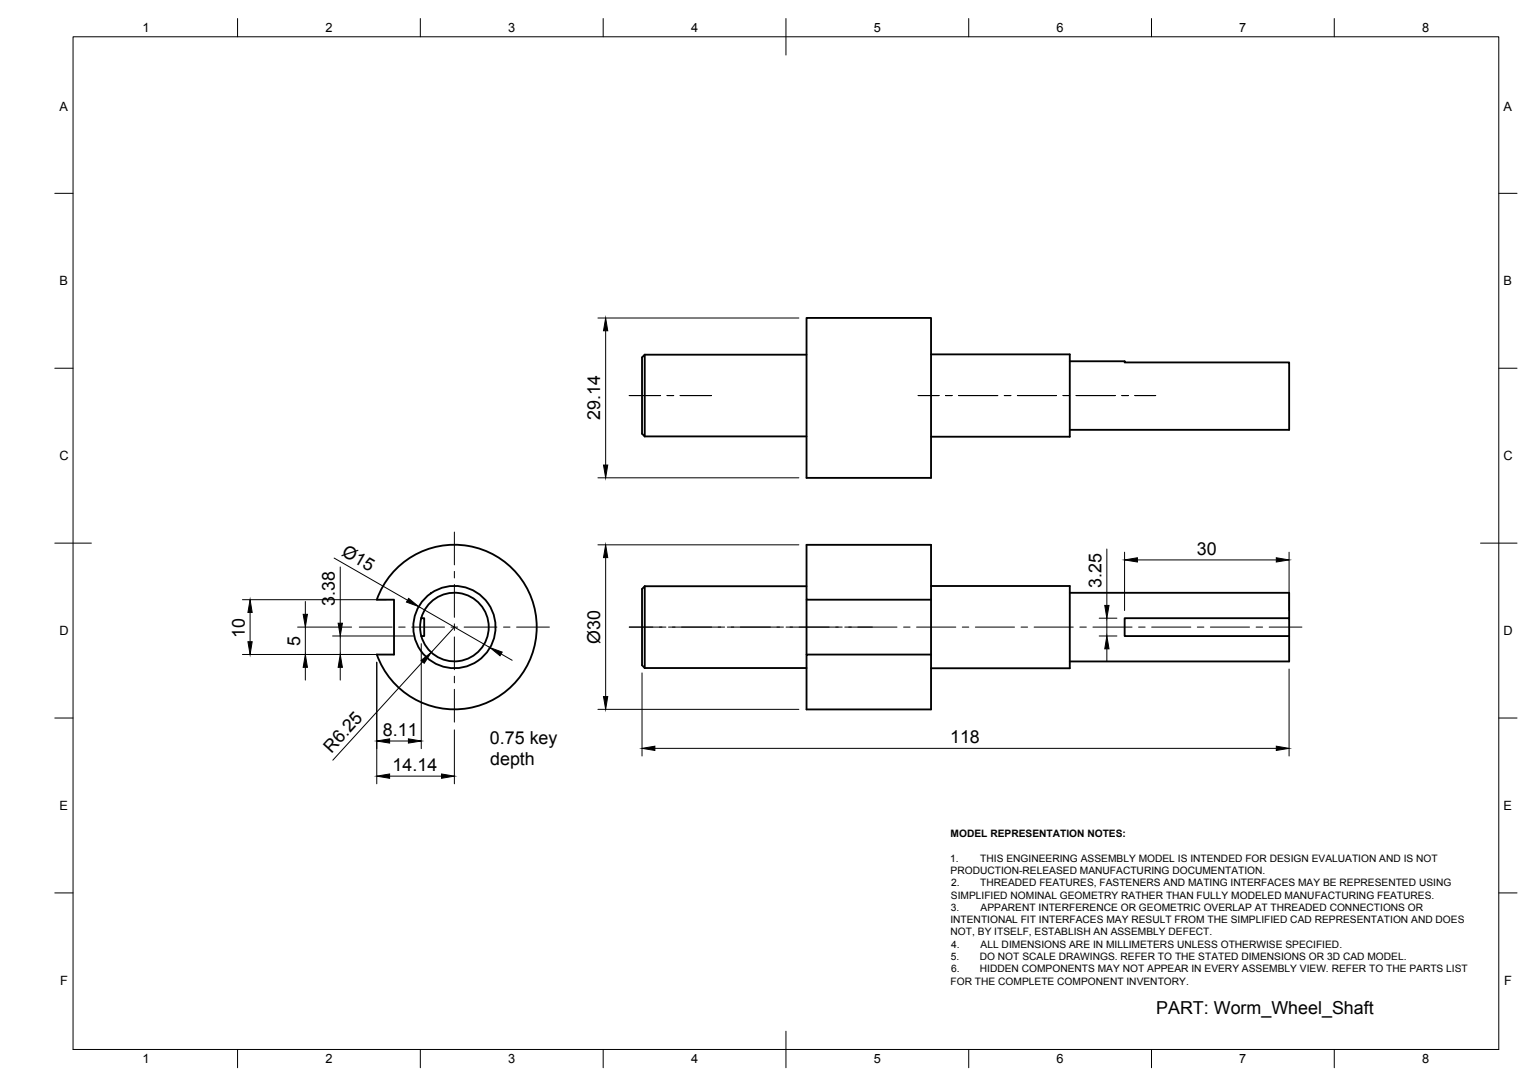
ISO-10303-21;
HEADER;
/* Generated by software containing ST-Developer
 * from STEP Tools, Inc. (www.steptools.com) 
 */

FILE_DESCRIPTION(
/* description */ ('STEP AP214'),
/* implementation_level */ '2;1');

FILE_NAME(
/* name */ 'Worm_Wheel_Shaft.step',
/* time_stamp */ '2026-10-05T13:15:56-07:00',
/* author */ (''),
/* organization */ (''),
/* preprocessor_version */ 'ST-DEVELOPER v20.2',
/* originating_system */ 'Autodesk Translation Framework v15.15.0.0',
/* authorisation */ '');

FILE_SCHEMA (('AUTOMOTIVE_DESIGN { 1 0 10303 214 3 1 1 }'));
ENDSEC;

DATA;
#10=MECHANICAL_DESIGN_GEOMETRIC_PRESENTATION_REPRESENTATION('',(#1347),#37881);
#593=CONICAL_SURFACE('',#11081,6.95000000000004,0.785398163397436);
#1323=SHAPE_REPRESENTATION_RELATIONSHIP('SRR','None',#37956,#1335);
#1335=ADVANCED_BREP_SHAPE_REPRESENTATION('',(#1359),#37871);
#1347=STYLED_ITEM('',(#38023),#1359);
#1359=MANIFOLD_SOLID_BREP('Body1',#10821);
#1402=FACE_BOUND('',#2276,.T.);
#1403=FACE_BOUND('',#2278,.T.);
#1404=FACE_BOUND('',#2280,.T.);
#1492=PLANE('',#11098);
#1493=PLANE('',#11099);
#1494=PLANE('',#11100);
#1495=PLANE('',#11101);
#1496=PLANE('',#11102);
#1497=PLANE('',#11103);
#1498=PLANE('',#11104);
#1499=PLANE('',#11105);
#1500=PLANE('',#11106);
#1501=PLANE('',#11107);
#1502=PLANE('',#11108);
#1503=PLANE('',#11109);
#1631=FACE_OUTER_BOUND('',#2265,.T.);
#1632=FACE_OUTER_BOUND('',#2266,.T.);
#1633=FACE_OUTER_BOUND('',#2267,.T.);
#1634=FACE_OUTER_BOUND('',#2268,.T.);
#1635=FACE_OUTER_BOUND('',#2269,.T.);
#1636=FACE_OUTER_BOUND('',#2270,.T.);
#1637=FACE_OUTER_BOUND('',#2271,.T.);
#1638=FACE_OUTER_BOUND('',#2272,.T.);
#1639=FACE_OUTER_BOUND('',#2273,.T.);
#1640=FACE_OUTER_BOUND('',#2274,.T.);
#1641=FACE_OUTER_BOUND('',#2275,.T.);
#1642=FACE_OUTER_BOUND('',#2277,.T.);
#1643=FACE_OUTER_BOUND('',#2279,.T.);
#1644=FACE_OUTER_BOUND('',#2281,.T.);
#1645=FACE_OUTER_BOUND('',#2282,.T.);
#1646=FACE_OUTER_BOUND('',#2283,.T.);
#1647=FACE_OUTER_BOUND('',#2284,.T.);
#2265=EDGE_LOOP('',(#7067,#7068,#7069,#7070,#7071));
#2266=EDGE_LOOP('',(#7072,#7073,#7074,#7075));
#2267=EDGE_LOOP('',(#7076,#7077,#7078,#7079));
#2268=EDGE_LOOP('',(#7080,#7081,#7082,#7083,#7084));
#2269=EDGE_LOOP('',(#7085,#7086,#7087,#7088,#7089,#7090,#7091,#7092));
#2270=EDGE_LOOP('',(#7093,#7094,#7095,#7096,#7097));
#2271=EDGE_LOOP('',(#7098));
#2272=EDGE_LOOP('',(#7099,#7100,#7101,#7102));
#2273=EDGE_LOOP('',(#7103,#7104,#7105,#7106));
#2274=EDGE_LOOP('',(#7107,#7108,#7109,#7110));
#2275=EDGE_LOOP('',(#7111,#7112,#7113,#7114));
#2276=EDGE_LOOP('',(#7115));
#2277=EDGE_LOOP('',(#7116,#7117,#7118,#7119));
#2278=EDGE_LOOP('',(#7120));
#2279=EDGE_LOOP('',(#7121));
#2280=EDGE_LOOP('',(#7122));
#2281=EDGE_LOOP('',(#7123,#7124,#7125,#7126));
#2282=EDGE_LOOP('',(#7127,#7128,#7129,#7130));
#2283=EDGE_LOOP('',(#7131,#7132,#7133,#7134));
#2284=EDGE_LOOP('',(#7135,#7136,#7137,#7138));
#2965=LINE('',#17230,#3266);
#2966=LINE('',#17236,#3267);
#2967=LINE('',#17243,#3268);
#2968=LINE('',#17246,#3269);
#2969=LINE('',#17249,#3270);
#2970=LINE('',#17255,#3271);
#2971=LINE('',#17259,#3272);
#2972=LINE('',#17263,#3273);
#2973=LINE('',#17268,#3274);
#2974=LINE('',#17269,#3275);
#2975=LINE('',#17270,#3276);
#2976=LINE('',#17274,#3277);
#2977=LINE('',#17276,#3278);
#2978=LINE('',#17277,#3279);
#2979=LINE('',#17280,#3280);
#2980=LINE('',#17282,#3281);
#2981=LINE('',#17283,#3282);
#2982=LINE('',#17285,#3283);
#2983=LINE('',#17286,#3284);
#2984=LINE('',#17292,#3285);
#2985=LINE('',#17294,#3286);
#2986=LINE('',#17295,#3287);
#2987=LINE('',#17297,#3288);
#2988=LINE('',#17299,#3289);
#3266=VECTOR('',#12224,6.95000000000004);
#3267=VECTOR('',#12231,7.5);
#3268=VECTOR('',#12238,1000.);
#3269=VECTOR('',#12241,1000.);
#3270=VECTOR('',#12244,7.45);
#3271=VECTOR('',#12251,6.25);
#3272=VECTOR('',#12254,1000.);
#3273=VECTOR('',#12257,1000.);
#3274=VECTOR('',#12262,1000.);
#3275=VECTOR('',#12263,1000.);
#3276=VECTOR('',#12264,1000.);
#3277=VECTOR('',#12269,1000.);
#3278=VECTOR('',#12270,1000.);
#3279=VECTOR('',#12271,1000.);
#3280=VECTOR('',#12274,1000.);
#3281=VECTOR('',#12275,1000.);
#3282=VECTOR('',#12276,1000.);
#3283=VECTOR('',#12279,1000.);
#3284=VECTOR('',#12280,1000.);
#3285=VECTOR('',#12289,1000.);
#3286=VECTOR('',#12290,1000.);
#3287=VECTOR('',#12291,1000.);
#3288=VECTOR('',#12294,1000.);
#3289=VECTOR('',#12297,1000.);
#3522=CIRCLE('',#11082,7.45);
#3523=CIRCLE('',#11083,7.45);
#3524=CIRCLE('',#11084,6.95000000000004);
#3525=CIRCLE('',#11086,7.5);
#3526=CIRCLE('',#11087,7.5);
#3527=CIRCLE('',#11089,15.);
#3528=CIRCLE('',#11090,15.);
#3529=CIRCLE('',#11092,7.45);
#3530=CIRCLE('',#11094,6.25);
#3531=CIRCLE('',#11095,6.25);
#3532=CIRCLE('',#11096,6.25);
#3533=CIRCLE('',#11097,6.25);
#4110=VERTEX_POINT('',#17225);
#4111=VERTEX_POINT('',#17226);
#4112=VERTEX_POINT('',#17229);
#4113=VERTEX_POINT('',#17233);
#4114=VERTEX_POINT('',#17235);
#4115=VERTEX_POINT('',#17239);
#4116=VERTEX_POINT('',#17240);
#4117=VERTEX_POINT('',#17242);
#4118=VERTEX_POINT('',#17244);
#4119=VERTEX_POINT('',#17248);
#4120=VERTEX_POINT('',#17252);
#4121=VERTEX_POINT('',#17254);
#4122=VERTEX_POINT('',#17256);
#4123=VERTEX_POINT('',#17258);
#4124=VERTEX_POINT('',#17260);
#4125=VERTEX_POINT('',#17262);
#4126=VERTEX_POINT('',#17266);
#4127=VERTEX_POINT('',#17267);
#4128=VERTEX_POINT('',#17273);
#4129=VERTEX_POINT('',#17275);
#4130=VERTEX_POINT('',#17279);
#4131=VERTEX_POINT('',#17281);
#4132=VERTEX_POINT('',#17291);
#4133=VERTEX_POINT('',#17293);
#5244=EDGE_CURVE('',#4110,#4111,#3522,.T.);
#5245=EDGE_CURVE('',#4111,#4110,#3523,.T.);
#5246=EDGE_CURVE('',#4111,#4112,#2965,.T.);
#5247=EDGE_CURVE('',#4112,#4112,#3524,.T.);
#5248=EDGE_CURVE('',#4113,#4113,#3525,.T.);
#5249=EDGE_CURVE('',#4113,#4114,#2966,.T.);
#5250=EDGE_CURVE('',#4114,#4114,#3526,.T.);
#5251=EDGE_CURVE('',#4115,#4116,#3527,.T.);
#5252=EDGE_CURVE('',#4115,#4117,#2967,.T.);
#5253=EDGE_CURVE('',#4117,#4118,#3528,.T.);
#5254=EDGE_CURVE('',#4116,#4118,#2968,.T.);
#5255=EDGE_CURVE('',#4110,#4119,#2969,.T.);
#5256=EDGE_CURVE('',#4119,#4119,#3529,.T.);
#5257=EDGE_CURVE('',#4120,#4120,#3530,.T.);
#5258=EDGE_CURVE('',#4120,#4121,#2970,.T.);
#5259=EDGE_CURVE('',#4122,#4121,#3531,.T.);
#5260=EDGE_CURVE('',#4123,#4122,#2971,.T.);
#5261=EDGE_CURVE('',#4124,#4123,#3532,.T.);
#5262=EDGE_CURVE('',#4124,#4125,#2972,.T.);
#5263=EDGE_CURVE('',#4121,#4125,#3533,.T.);
#5264=EDGE_CURVE('',#4126,#4127,#2973,.T.);
#5265=EDGE_CURVE('',#4126,#4122,#2974,.T.);
#5266=EDGE_CURVE('',#4127,#4125,#2975,.T.);
#5267=EDGE_CURVE('',#4128,#4117,#2976,.T.);
#5268=EDGE_CURVE('',#4129,#4115,#2977,.T.);
#5269=EDGE_CURVE('',#4129,#4128,#2978,.T.);
#5270=EDGE_CURVE('',#4130,#4118,#2979,.T.);
#5271=EDGE_CURVE('',#4131,#4130,#2980,.T.);
#5272=EDGE_CURVE('',#4131,#4116,#2981,.T.);
#5273=EDGE_CURVE('',#4128,#4130,#2982,.T.);
#5274=EDGE_CURVE('',#4129,#4131,#2983,.T.);
#5275=EDGE_CURVE('',#4132,#4123,#2984,.T.);
#5276=EDGE_CURVE('',#4132,#4133,#2985,.T.);
#5277=EDGE_CURVE('',#4133,#4124,#2986,.T.);
#5278=EDGE_CURVE('',#4132,#4126,#2987,.T.);
#5279=EDGE_CURVE('',#4133,#4127,#2988,.T.);
#7067=ORIENTED_EDGE('',*,*,#5244,.F.);
#7068=ORIENTED_EDGE('',*,*,#5245,.F.);
#7069=ORIENTED_EDGE('',*,*,#5246,.T.);
#7070=ORIENTED_EDGE('',*,*,#5247,.F.);
#7071=ORIENTED_EDGE('',*,*,#5246,.F.);
#7072=ORIENTED_EDGE('',*,*,#5248,.T.);
#7073=ORIENTED_EDGE('',*,*,#5249,.T.);
#7074=ORIENTED_EDGE('',*,*,#5250,.F.);
#7075=ORIENTED_EDGE('',*,*,#5249,.F.);
#7076=ORIENTED_EDGE('',*,*,#5251,.F.);
#7077=ORIENTED_EDGE('',*,*,#5252,.T.);
#7078=ORIENTED_EDGE('',*,*,#5253,.T.);
#7079=ORIENTED_EDGE('',*,*,#5254,.F.);
#7080=ORIENTED_EDGE('',*,*,#5244,.T.);
#7081=ORIENTED_EDGE('',*,*,#5245,.T.);
#7082=ORIENTED_EDGE('',*,*,#5255,.T.);
#7083=ORIENTED_EDGE('',*,*,#5256,.T.);
#7084=ORIENTED_EDGE('',*,*,#5255,.F.);
#7085=ORIENTED_EDGE('',*,*,#5257,.T.);
#7086=ORIENTED_EDGE('',*,*,#5258,.T.);
#7087=ORIENTED_EDGE('',*,*,#5259,.F.);
#7088=ORIENTED_EDGE('',*,*,#5260,.F.);
#7089=ORIENTED_EDGE('',*,*,#5261,.F.);
#7090=ORIENTED_EDGE('',*,*,#5262,.T.);
#7091=ORIENTED_EDGE('',*,*,#5263,.F.);
#7092=ORIENTED_EDGE('',*,*,#5258,.F.);
#7093=ORIENTED_EDGE('',*,*,#5264,.F.);
#7094=ORIENTED_EDGE('',*,*,#5265,.T.);
#7095=ORIENTED_EDGE('',*,*,#5259,.T.);
#7096=ORIENTED_EDGE('',*,*,#5263,.T.);
#7097=ORIENTED_EDGE('',*,*,#5266,.F.);
#7098=ORIENTED_EDGE('',*,*,#5247,.T.);
#7099=ORIENTED_EDGE('',*,*,#5267,.T.);
#7100=ORIENTED_EDGE('',*,*,#5252,.F.);
#7101=ORIENTED_EDGE('',*,*,#5268,.F.);
#7102=ORIENTED_EDGE('',*,*,#5269,.T.);
#7103=ORIENTED_EDGE('',*,*,#5270,.F.);
#7104=ORIENTED_EDGE('',*,*,#5271,.F.);
#7105=ORIENTED_EDGE('',*,*,#5272,.T.);
#7106=ORIENTED_EDGE('',*,*,#5254,.T.);
#7107=ORIENTED_EDGE('',*,*,#5273,.F.);
#7108=ORIENTED_EDGE('',*,*,#5269,.F.);
#7109=ORIENTED_EDGE('',*,*,#5274,.T.);
#7110=ORIENTED_EDGE('',*,*,#5271,.T.);
#7111=ORIENTED_EDGE('',*,*,#5268,.T.);
#7112=ORIENTED_EDGE('',*,*,#5251,.T.);
#7113=ORIENTED_EDGE('',*,*,#5272,.F.);
#7114=ORIENTED_EDGE('',*,*,#5274,.F.);
#7115=ORIENTED_EDGE('',*,*,#5248,.F.);
#7116=ORIENTED_EDGE('',*,*,#5267,.F.);
#7117=ORIENTED_EDGE('',*,*,#5273,.T.);
#7118=ORIENTED_EDGE('',*,*,#5270,.T.);
#7119=ORIENTED_EDGE('',*,*,#5253,.F.);
#7120=ORIENTED_EDGE('',*,*,#5256,.F.);
#7121=ORIENTED_EDGE('',*,*,#5250,.T.);
#7122=ORIENTED_EDGE('',*,*,#5257,.F.);
#7123=ORIENTED_EDGE('',*,*,#5261,.T.);
#7124=ORIENTED_EDGE('',*,*,#5275,.F.);
#7125=ORIENTED_EDGE('',*,*,#5276,.T.);
#7126=ORIENTED_EDGE('',*,*,#5277,.T.);
#7127=ORIENTED_EDGE('',*,*,#5260,.T.);
#7128=ORIENTED_EDGE('',*,*,#5265,.F.);
#7129=ORIENTED_EDGE('',*,*,#5278,.F.);
#7130=ORIENTED_EDGE('',*,*,#5275,.T.);
#7131=ORIENTED_EDGE('',*,*,#5277,.F.);
#7132=ORIENTED_EDGE('',*,*,#5279,.T.);
#7133=ORIENTED_EDGE('',*,*,#5266,.T.);
#7134=ORIENTED_EDGE('',*,*,#5262,.F.);
#7135=ORIENTED_EDGE('',*,*,#5264,.T.);
#7136=ORIENTED_EDGE('',*,*,#5279,.F.);
#7137=ORIENTED_EDGE('',*,*,#5276,.F.);
#7138=ORIENTED_EDGE('',*,*,#5278,.T.);
#10061=CYLINDRICAL_SURFACE('',#11085,7.5);
#10062=CYLINDRICAL_SURFACE('',#11088,15.);
#10063=CYLINDRICAL_SURFACE('',#11091,7.45);
#10064=CYLINDRICAL_SURFACE('',#11093,6.25);
#10276=ADVANCED_FACE('',(#1631),#593,.T.);
#10277=ADVANCED_FACE('',(#1632),#10061,.T.);
#10278=ADVANCED_FACE('',(#1633),#10062,.T.);
#10279=ADVANCED_FACE('',(#1634),#10063,.T.);
#10280=ADVANCED_FACE('',(#1635),#10064,.T.);
#10281=ADVANCED_FACE('',(#1636),#1492,.T.);
#10282=ADVANCED_FACE('',(#1637),#1493,.T.);
#10283=ADVANCED_FACE('',(#1638),#1494,.F.);
#10284=ADVANCED_FACE('',(#1639),#1495,.T.);
#10285=ADVANCED_FACE('',(#1640),#1496,.T.);
#10286=ADVANCED_FACE('',(#1641,#1402),#1497,.T.);
#10287=ADVANCED_FACE('',(#1642,#1403),#1498,.F.);
#10288=ADVANCED_FACE('',(#1643,#1404),#1499,.T.);
#10289=ADVANCED_FACE('',(#1644),#1500,.T.);
#10290=ADVANCED_FACE('',(#1645),#1501,.T.);
#10291=ADVANCED_FACE('',(#1646),#1502,.F.);
#10292=ADVANCED_FACE('',(#1647),#1503,.F.);
#10821=CLOSED_SHELL('',(#10276,#10277,#10278,#10279,#10280,#10281,#10282,
#10283,#10284,#10285,#10286,#10287,#10288,#10289,#10290,#10291,#10292));
#11080=AXIS2_PLACEMENT_3D('',#17223,#12216,#12217);
#11081=AXIS2_PLACEMENT_3D('',#17224,#12218,#12219);
#11082=AXIS2_PLACEMENT_3D('',#17227,#12220,#12221);
#11083=AXIS2_PLACEMENT_3D('',#17228,#12222,#12223);
#11084=AXIS2_PLACEMENT_3D('',#17231,#12225,#12226);
#11085=AXIS2_PLACEMENT_3D('',#17232,#12227,#12228);
#11086=AXIS2_PLACEMENT_3D('',#17234,#12229,#12230);
#11087=AXIS2_PLACEMENT_3D('',#17237,#12232,#12233);
#11088=AXIS2_PLACEMENT_3D('',#17238,#12234,#12235);
#11089=AXIS2_PLACEMENT_3D('',#17241,#12236,#12237);
#11090=AXIS2_PLACEMENT_3D('',#17245,#12239,#12240);
#11091=AXIS2_PLACEMENT_3D('',#17247,#12242,#12243);
#11092=AXIS2_PLACEMENT_3D('',#17250,#12245,#12246);
#11093=AXIS2_PLACEMENT_3D('',#17251,#12247,#12248);
#11094=AXIS2_PLACEMENT_3D('',#17253,#12249,#12250);
#11095=AXIS2_PLACEMENT_3D('',#17257,#12252,#12253);
#11096=AXIS2_PLACEMENT_3D('',#17261,#12255,#12256);
#11097=AXIS2_PLACEMENT_3D('',#17264,#12258,#12259);
#11098=AXIS2_PLACEMENT_3D('',#17265,#12260,#12261);
#11099=AXIS2_PLACEMENT_3D('',#17271,#12265,#12266);
#11100=AXIS2_PLACEMENT_3D('',#17272,#12267,#12268);
#11101=AXIS2_PLACEMENT_3D('',#17278,#12272,#12273);
#11102=AXIS2_PLACEMENT_3D('',#17284,#12277,#12278);
#11103=AXIS2_PLACEMENT_3D('',#17287,#12281,#12282);
#11104=AXIS2_PLACEMENT_3D('',#17288,#12283,#12284);
#11105=AXIS2_PLACEMENT_3D('',#17289,#12285,#12286);
#11106=AXIS2_PLACEMENT_3D('',#17290,#12287,#12288);
#11107=AXIS2_PLACEMENT_3D('',#17296,#12292,#12293);
#11108=AXIS2_PLACEMENT_3D('',#17298,#12295,#12296);
#11109=AXIS2_PLACEMENT_3D('',#17300,#12298,#12299);
#12216=DIRECTION('axis',(0.,0.,1.));
#12217=DIRECTION('refdir',(1.,0.,0.));
#12218=DIRECTION('center_axis',(1.,0.,5.91645678915759E-31));
#12219=DIRECTION('ref_axis',(5.91645678915759E-31,-1.28868988380477E-29,
-1.));
#12220=DIRECTION('center_axis',(1.,0.,5.91645678915759E-31));
#12221=DIRECTION('ref_axis',(-5.91645678915759E-31,1.29257043247465E-29,
1.));
#12222=DIRECTION('center_axis',(1.,0.,5.91645678915759E-31));
#12223=DIRECTION('ref_axis',(-5.91645678915759E-31,1.29257043247465E-29,
1.));
#12224=DIRECTION('',(-0.707106781186556,8.65956056235392E-17,-0.707106781186539));
#12225=DIRECTION('center_axis',(-1.,0.,-5.91645678915759E-31));
#12226=DIRECTION('ref_axis',(-5.91645678915759E-31,1.28868988380477E-29,
1.));
#12227=DIRECTION('center_axis',(-1.,0.,-5.91645678915759E-31));
#12228=DIRECTION('ref_axis',(-5.91645678915759E-31,1.29422492262822E-29,
1.));
#12229=DIRECTION('center_axis',(1.,0.,5.91645678915759E-31));
#12230=DIRECTION('ref_axis',(5.91645678915759E-31,-1.29422492262822E-29,
-1.));
#12231=DIRECTION('',(1.,0.,5.91645678915759E-31));
#12232=DIRECTION('center_axis',(1.,0.,5.91645678915759E-31));
#12233=DIRECTION('ref_axis',(5.91645678915759E-31,-1.29422492262822E-29,
-1.));
#12234=DIRECTION('center_axis',(-1.,0.,-5.91645678915759E-31));
#12235=DIRECTION('ref_axis',(7.00649232162409E-46,-1.,-1.07187543957222E-15));
#12236=DIRECTION('center_axis',(1.,0.,5.91645678915759E-31));
#12237=DIRECTION('ref_axis',(5.91645678915759E-31,-1.28395329625816E-29,
-1.));
#12238=DIRECTION('',(-1.,0.,-5.91645678915759E-31));
#12239=DIRECTION('center_axis',(1.,0.,5.91645678915759E-31));
#12240=DIRECTION('ref_axis',(5.91645678915759E-31,-1.28395329625816E-29,
-1.));
#12241=DIRECTION('',(-1.,0.,-5.91645678915759E-31));
#12242=DIRECTION('center_axis',(-1.,0.,-5.91645678915759E-31));
#12243=DIRECTION('ref_axis',(-5.91645678915759E-31,1.28868988380477E-29,
1.));
#12244=DIRECTION('',(1.,0.,5.91645678915759E-31));
#12245=DIRECTION('center_axis',(-1.,0.,-5.91645678915759E-31));
#12246=DIRECTION('ref_axis',(-5.91645678915759E-31,1.29257043247465E-29,
1.));
#12247=DIRECTION('center_axis',(-1.,0.,-5.91645678915759E-31));
#12248=DIRECTION('ref_axis',(-5.91645678915759E-31,1.28868988380477E-29,
1.));
#12249=DIRECTION('center_axis',(1.,0.,5.91645678915759E-31));
#12250=DIRECTION('ref_axis',(5.91645678915759E-31,-1.28189897098414E-29,
-1.));
#12251=DIRECTION('',(1.,0.,5.91645678915759E-31));
#12252=DIRECTION('center_axis',(1.,0.,5.91645678915759E-31));
#12253=DIRECTION('ref_axis',(5.91645678915759E-31,-1.28868988380477E-29,
-1.));
#12254=DIRECTION('',(1.,0.,5.91645678915759E-31));
#12255=DIRECTION('center_axis',(1.,0.,5.91645678915759E-31));
#12256=DIRECTION('ref_axis',(5.91645678915759E-31,-1.28189897098414E-29,
-1.));
#12257=DIRECTION('',(1.,0.,5.91645678915759E-31));
#12258=DIRECTION('center_axis',(1.,0.,5.91645678915759E-31));
#12259=DIRECTION('ref_axis',(5.91645678915759E-31,-1.28868988380477E-29,
-1.));
#12260=DIRECTION('center_axis',(1.,-1.52489560243109E-59,-5.91645678915759E-31));
#12261=DIRECTION('ref_axis',(-5.91645678915759E-31,-1.28868988380477E-29,
-1.));
#12262=DIRECTION('',(-3.94430452610506E-31,2.22044604925018E-16,-1.));
#12263=DIRECTION('',(0.,1.,1.28868988380477E-29));
#12264=DIRECTION('',(0.,1.,1.28868988380477E-29));
#12265=DIRECTION('center_axis',(-1.,1.52489560243109E-59,5.91645678915759E-31));
#12266=DIRECTION('ref_axis',(5.91645678915759E-31,1.28868988380477E-29,
1.));
#12267=DIRECTION('center_axis',(-5.91645678915759E-31,1.28868988380477E-29,
1.));
#12268=DIRECTION('ref_axis',(1.,5.52714787526044E-76,5.91645678915759E-31));
#12269=DIRECTION('',(0.,1.,1.28868988380477E-29));
#12270=DIRECTION('',(0.,1.,1.28868988380477E-29));
#12271=DIRECTION('',(-1.,0.,-5.91645678915759E-31));
#12272=DIRECTION('center_axis',(-5.91645678915759E-31,1.28868988380477E-29,
1.));
#12273=DIRECTION('ref_axis',(1.,5.52714787526044E-76,5.91645678915759E-31));
#12274=DIRECTION('',(0.,1.,1.28868988380477E-29));
#12275=DIRECTION('',(-1.,0.,-5.91645678915759E-31));
#12276=DIRECTION('',(0.,1.,1.28868988380477E-29));
#12277=DIRECTION('center_axis',(-1.52489560243109E-59,1.,-1.28868988380477E-29));
#12278=DIRECTION('ref_axis',(5.91645678915759E-31,1.28868988380477E-29,
1.));
#12279=DIRECTION('',(-5.91645678915759E-31,-1.28868988380477E-29,-1.));
#12280=DIRECTION('',(-5.91645678915759E-31,-1.28868988380477E-29,-1.));
#12281=DIRECTION('center_axis',(1.,-1.52489560243109E-59,-5.91645678915759E-31));
#12282=DIRECTION('ref_axis',(-5.91645678915759E-31,-1.28868988380477E-29,
-1.));
#12283=DIRECTION('center_axis',(1.,-1.52489560243109E-59,-5.91645678915759E-31));
#12284=DIRECTION('ref_axis',(-5.91645678915759E-31,-1.28868988380477E-29,
-1.));
#12285=DIRECTION('center_axis',(1.,-1.52489560243109E-59,-5.91645678915759E-31));
#12286=DIRECTION('ref_axis',(-5.91645678915759E-31,-1.28868988380477E-29,
-1.));
#12287=DIRECTION('center_axis',(1.,-1.52489560243109E-59,-5.91645678915759E-31));
#12288=DIRECTION('ref_axis',(-5.91645678915759E-31,-1.28868988380477E-29,
-1.));
#12289=DIRECTION('',(0.,1.,1.28868988380477E-29));
#12290=DIRECTION('',(-3.94430452610506E-31,2.22044604925018E-16,-1.));
#12291=DIRECTION('',(0.,1.,1.28868988380477E-29));
#12292=DIRECTION('center_axis',(5.91645678915759E-31,-1.28868988380477E-29,
-1.));
#12293=DIRECTION('ref_axis',(-1.,-5.52714787526044E-76,-5.91645678915759E-31));
#12294=DIRECTION('',(1.,0.,5.91645678915759E-31));
#12295=DIRECTION('center_axis',(5.91645678915759E-31,-1.28868988380477E-29,
-1.));
#12296=DIRECTION('ref_axis',(-1.,-5.52714787526044E-76,-5.91645678915759E-31));
#12297=DIRECTION('',(1.,0.,5.91645678915759E-31));
#12298=DIRECTION('center_axis',(1.01610171333826E-59,-1.,-2.22044604925018E-16));
#12299=DIRECTION('ref_axis',(-3.94430452610506E-31,2.22044604925018E-16,
-1.));
#17223=CARTESIAN_POINT('',(0.,0.,0.));
#17224=CARTESIAN_POINT('Origin',(0.,0.,0.));
#17225=CARTESIAN_POINT('',(0.499999999999973,9.12361865364679E-16,-7.45));
#17226=CARTESIAN_POINT('',(0.499999999999979,-9.12361865364683E-16,7.45000000000001));
#17227=CARTESIAN_POINT('Origin',(0.499999999999973,-6.93889390390723E-15,
5.20417042793042E-15));
#17228=CARTESIAN_POINT('Origin',(0.499999999999973,-6.93889390390723E-15,
5.20417042793042E-15));
#17229=CARTESIAN_POINT('',(-2.67390226427335E-16,-8.51129525407326E-16,
6.95000000000004));
#17230=CARTESIAN_POINT('',(-4.11193746846455E-30,-8.51129525407326E-16,
6.95000000000004));
#17231=CARTESIAN_POINT('Origin',(0.,0.,0.));
#17232=CARTESIAN_POINT('Origin',(78.,-8.67361737988404E-15,6.93889390390723E-15));
#17233=CARTESIAN_POINT('',(52.7,-9.59210247924465E-15,-7.49999999999999));
#17234=CARTESIAN_POINT('Origin',(52.7,-8.67361737988404E-15,6.93889390390723E-15));
#17235=CARTESIAN_POINT('',(78.,-9.59210247924465E-15,-7.49999999999999));
#17236=CARTESIAN_POINT('',(78.,-9.59210247924465E-15,-7.49999999999999));
#17237=CARTESIAN_POINT('Origin',(78.,-8.67361737988404E-15,6.93889390390723E-15));
#17238=CARTESIAN_POINT('Origin',(52.7,-8.67361737988404E-15,6.93889390390723E-15));
#17239=CARTESIAN_POINT('',(52.7,14.1421356237309,5.00000000000001));
#17240=CARTESIAN_POINT('',(52.7,14.1421356237309,-4.99999999999999));
#17241=CARTESIAN_POINT('Origin',(52.7,-8.67361737988404E-15,6.93889390390723E-15));
#17242=CARTESIAN_POINT('',(30.,14.1421356237309,5.00000000000001));
#17243=CARTESIAN_POINT('',(52.7,14.1421356237309,5.00000000000001));
#17244=CARTESIAN_POINT('',(30.,14.142135623731,-4.99999999999999));
#17245=CARTESIAN_POINT('Origin',(30.,-6.93889390390723E-15,6.93889390390723E-15));
#17246=CARTESIAN_POINT('',(52.7,14.1421356237309,-4.99999999999999));
#17247=CARTESIAN_POINT('Origin',(0.,0.,0.));
#17248=CARTESIAN_POINT('',(30.,-9.12361865364874E-16,-7.45));
#17249=CARTESIAN_POINT('',(4.4077603079224E-30,-9.12361865364874E-16,-7.45));
#17250=CARTESIAN_POINT('Origin',(30.,-6.93889390390723E-15,6.93889390390723E-15));
#17251=CARTESIAN_POINT('Origin',(118.,0.,0.));
#17252=CARTESIAN_POINT('',(78.,-7.65404249467176E-16,-6.25));
#17253=CARTESIAN_POINT('Origin',(78.,-8.67361737988404E-15,6.93889390390723E-15));
#17254=CARTESIAN_POINT('',(118.,-7.65404249467176E-16,-6.25));
#17255=CARTESIAN_POINT('',(118.,-7.65404249467176E-16,-6.25));
#17256=CARTESIAN_POINT('',(118.,6.03505385228666,1.625));
#17257=CARTESIAN_POINT('Origin',(118.,0.,0.));
#17258=CARTESIAN_POINT('',(88.,6.03505385228665,1.625));
#17259=CARTESIAN_POINT('',(118.,6.03505385228666,1.625));
#17260=CARTESIAN_POINT('',(88.,6.03505385228665,-1.625));
#17261=CARTESIAN_POINT('Origin',(88.,-6.93889390390723E-15,3.46944695195361E-15));
#17262=CARTESIAN_POINT('',(118.,6.03505385228666,-1.625));
#17263=CARTESIAN_POINT('',(118.,6.03505385228666,-1.625));
#17264=CARTESIAN_POINT('Origin',(118.,0.,0.));
#17265=CARTESIAN_POINT('Origin',(118.,0.,0.));
#17266=CARTESIAN_POINT('',(118.,5.5,1.625));
#17267=CARTESIAN_POINT('',(118.,5.5,-1.62499999999999));
#17268=CARTESIAN_POINT('',(118.,5.5,0.));
#17269=CARTESIAN_POINT('',(118.,-3.46944695195361E-15,1.625));
#17270=CARTESIAN_POINT('',(118.,-1.73472347597681E-15,-1.625));
#17271=CARTESIAN_POINT('Origin',(0.,0.,0.));
#17272=CARTESIAN_POINT('Origin',(52.7,-5.20417042793042E-15,5.00000000000001));
#17273=CARTESIAN_POINT('',(30.,11.,5.00000000000001));
#17274=CARTESIAN_POINT('',(30.,-6.93889390390723E-15,5.00000000000001));
#17275=CARTESIAN_POINT('',(52.7,11.,5.00000000000001));
#17276=CARTESIAN_POINT('',(52.7,-5.20417042793042E-15,5.00000000000001));
#17277=CARTESIAN_POINT('',(52.7,11.,5.00000000000001));
#17278=CARTESIAN_POINT('Origin',(52.7,-5.20417042793042E-15,-4.99999999999999));
#17279=CARTESIAN_POINT('',(30.,11.,-4.99999999999999));
#17280=CARTESIAN_POINT('',(30.,-5.20417042793042E-15,-4.99999999999999));
#17281=CARTESIAN_POINT('',(52.7,11.,-4.99999999999999));
#17282=CARTESIAN_POINT('',(52.7,11.,-4.99999999999999));
#17283=CARTESIAN_POINT('',(52.7,-5.20417042793042E-15,-4.99999999999999));
#17284=CARTESIAN_POINT('Origin',(52.7,11.,5.20417042793042E-15));
#17285=CARTESIAN_POINT('',(30.,11.,6.93889390390723E-15));
#17286=CARTESIAN_POINT('',(52.7,11.,5.20417042793042E-15));
#17287=CARTESIAN_POINT('Origin',(52.7,-8.67361737988404E-15,6.93889390390723E-15));
#17288=CARTESIAN_POINT('Origin',(30.,-6.93889390390723E-15,6.93889390390723E-15));
#17289=CARTESIAN_POINT('Origin',(78.,-8.67361737988404E-15,6.93889390390723E-15));
#17290=CARTESIAN_POINT('Origin',(88.,-6.93889390390723E-15,3.46944695195361E-15));
#17291=CARTESIAN_POINT('',(88.,5.49999999999999,1.625));
#17292=CARTESIAN_POINT('',(88.,-5.20417042793042E-15,1.625));
#17293=CARTESIAN_POINT('',(88.,5.5,-1.62499999999999));
#17294=CARTESIAN_POINT('',(88.,5.5,0.));
#17295=CARTESIAN_POINT('',(88.,-6.93889390390723E-15,-1.62499999999999));
#17296=CARTESIAN_POINT('Origin',(88.,-5.20417042793042E-15,1.625));
#17297=CARTESIAN_POINT('',(88.,5.49999999999999,1.625));
#17298=CARTESIAN_POINT('Origin',(88.,-6.93889390390723E-15,-1.62499999999999));
#17299=CARTESIAN_POINT('',(88.,5.5,-1.62499999999999));
#17300=CARTESIAN_POINT('Origin',(88.,5.5,0.));
#37857=UNCERTAINTY_MEASURE_WITH_UNIT(LENGTH_MEASURE(0.01),#37882,
'DISTANCE_ACCURACY_VALUE',
'Maximum model space distance between geometric entities at asserted c
onnectivities');
#37867=UNCERTAINTY_MEASURE_WITH_UNIT(LENGTH_MEASURE(0.01),#37882,
'DISTANCE_ACCURACY_VALUE',
'Maximum model space distance between geometric entities at asserted c
onnectivities');
#37871=(
GEOMETRIC_REPRESENTATION_CONTEXT(3)
GLOBAL_UNCERTAINTY_ASSIGNED_CONTEXT((#37857))
GLOBAL_UNIT_ASSIGNED_CONTEXT((#37882,#37884,#37885))
REPRESENTATION_CONTEXT('','3D')
);
#37881=(
GEOMETRIC_REPRESENTATION_CONTEXT(3)
GLOBAL_UNCERTAINTY_ASSIGNED_CONTEXT((#37867))
GLOBAL_UNIT_ASSIGNED_CONTEXT((#37882,#37884,#37885))
REPRESENTATION_CONTEXT('','3D')
);
#37882=(
LENGTH_UNIT()
NAMED_UNIT(*)
SI_UNIT(.MILLI.,.METRE.)
);
#37884=(
NAMED_UNIT(*)
PLANE_ANGLE_UNIT()
SI_UNIT($,.RADIAN.)
);
#37885=(
NAMED_UNIT(*)
SI_UNIT($,.STERADIAN.)
SOLID_ANGLE_UNIT()
);
#37889=SHAPE_DEFINITION_REPRESENTATION(#37902,#37956);
#37902=PRODUCT_DEFINITION_SHAPE('',$,#37970);
#37956=SHAPE_REPRESENTATION('',(#11080),#37871);
#37966=PRODUCT_DEFINITION_CONTEXT('part definition',#38007,'design');
#37970=PRODUCT_DEFINITION('PS03','Worm_Wheel_Shaft',#37983,#37966);
#37983=PRODUCT_DEFINITION_FORMATION('',$,#38012);
#38007=APPLICATION_CONTEXT(
'Core Data for Automotive Mechanical Design Process');
#38008=PRODUCT_CONTEXT('part definition',#38007,'mechanical');
#38012=PRODUCT('PS03','Worm_Wheel_Shaft',$,(#38008));
#38023=PRESENTATION_STYLE_ASSIGNMENT((#38025));
#38025=SURFACE_STYLE_USAGE(.BOTH.,#38027);
#38027=SURFACE_SIDE_STYLE('',(#38029));
#38029=SURFACE_STYLE_FILL_AREA(#38031);
#38031=FILL_AREA_STYLE('Opaque(202,209,238)',(#38033));
#38033=FILL_AREA_STYLE_COLOUR('Opaque(202,209,238)',#38035);
#38035=COLOUR_RGB('Opaque(202,209,238)', 0.66274510, 0.83137255, 0.94901961);
ENDSEC;
END-ISO-10303-21;
